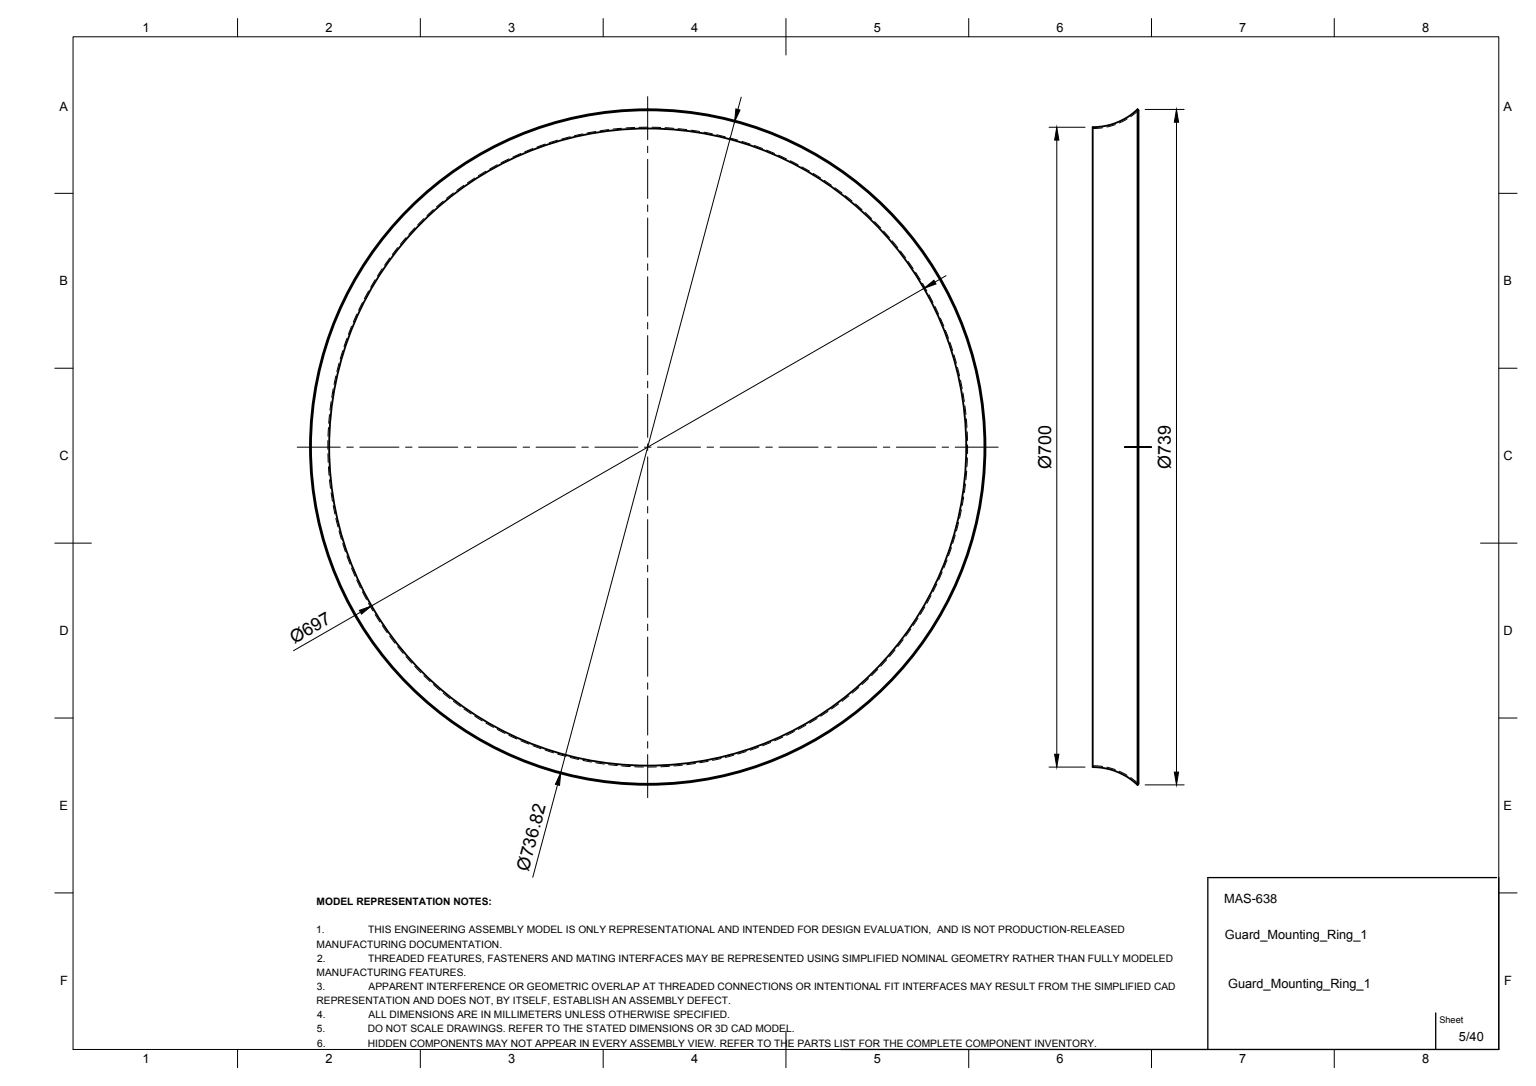
ISO-10303-21;
HEADER;
FILE_DESCRIPTION((''),'2;1');
FILE_NAME('Guard_Mounting_Ring_1.step','2026-10-09T12:00:21-07:00',(''),(''),'','','');
FILE_SCHEMA (('AUTOMOTIVE_DESIGN { 1 0 10303 214 3 1 1 }'));
ENDSEC;
DATA;
#10=MECHANICAL_DESIGN_GEOMETRIC_PRESENTATION_REPRESENTATION('',(#396),#10334);
#332=SHAPE_REPRESENTATION_RELATIONSHIP('SRR','None',#10448,#364) ;
#364=ADVANCED_BREP_SHAPE_REPRESENTATION('',(#436),#10300) ;
#396=STYLED_ITEM('',(#10631),#436) ;
#436=MANIFOLD_SOLID_BREP('Body1',#3558) ;
#468=FACE_BOUND('',#1054,.T.) ;
#477=PLANE('',#3957) ;
#532=LINE('',#5624,#690) ;
#690=VECTOR('',#4472,36.8410607518303) ;
#848=CONICAL_SURFACE('',#3956,36.8410607518303,0.812867971023228) ;
#851=FACE_OUTER_BOUND('',#1050,.T.) ;
#852=FACE_OUTER_BOUND('',#1051,.T.) ;
#853=FACE_OUTER_BOUND('',#1052,.T.) ;
#854=FACE_OUTER_BOUND('',#1053,.T.) ;
#1050=EDGE_LOOP('',(#2307,#2308,#2309,#2310,#2311)) ;
#1051=EDGE_LOOP('',(#2312,#2313,#2314,#2315,#2316)) ;
#1052=EDGE_LOOP('',(#2317,#2318,#2319,#2320,#2321,#2322)) ;
#1053=EDGE_LOOP('',(#2323)) ;
#1054=EDGE_LOOP('',(#2324)) ;
#1258=CIRCLE('',#3947,36.9499999999999) ;
#1259=CIRCLE('',#3948,36.9499999999999) ;
#1260=CIRCLE('',#3949,7.1235909466484) ;
#1261=CIRCLE('',#3950,35.) ;
#1262=CIRCLE('',#3952,34.8499999999999) ;
#1263=CIRCLE('',#3953,7.27359094664848) ;
#1264=CIRCLE('',#3954,36.8410607518303) ;
#1265=CIRCLE('',#3955,36.8410607518303) ;
#1499=VERTEX_POINT('',#5608) ;
#1500=VERTEX_POINT('',#5609) ;
#1501=VERTEX_POINT('',#5612) ;
#1502=VERTEX_POINT('',#5616) ;
#1503=VERTEX_POINT('',#5618) ;
#1504=VERTEX_POINT('',#5620) ;
#1810=EDGE_CURVE('',#1499,#1500,#1258,.T.) ;
#1811=EDGE_CURVE('',#1500,#1499,#1259,.T.) ;
#1812=EDGE_CURVE('',#1500,#1501,#1260,.T.) ;
#1813=EDGE_CURVE('',#1501,#1501,#1261,.T.) ;
#1814=EDGE_CURVE('',#1502,#1502,#1262,.T.) ;
#1815=EDGE_CURVE('',#1502,#1503,#1263,.T.) ;
#1816=EDGE_CURVE('',#1503,#1504,#1264,.T.) ;
#1817=EDGE_CURVE('',#1504,#1503,#1265,.T.) ;
#1818=EDGE_CURVE('',#1499,#1504,#532,.T.) ;
#2307=ORIENTED_EDGE('',*,*,#1810,.F.) ;
#2308=ORIENTED_EDGE('',*,*,#1811,.F.) ;
#2309=ORIENTED_EDGE('',*,*,#1812,.T.) ;
#2310=ORIENTED_EDGE('',*,*,#1813,.T.) ;
#2311=ORIENTED_EDGE('',*,*,#1812,.F.) ;
#2312=ORIENTED_EDGE('',*,*,#1814,.F.) ;
#2313=ORIENTED_EDGE('',*,*,#1815,.T.) ;
#2314=ORIENTED_EDGE('',*,*,#1816,.T.) ;
#2315=ORIENTED_EDGE('',*,*,#1817,.T.) ;
#2316=ORIENTED_EDGE('',*,*,#1815,.F.) ;
#2317=ORIENTED_EDGE('',*,*,#1810,.T.) ;
#2318=ORIENTED_EDGE('',*,*,#1811,.T.) ;
#2319=ORIENTED_EDGE('',*,*,#1818,.T.) ;
#2320=ORIENTED_EDGE('',*,*,#1816,.F.) ;
#2321=ORIENTED_EDGE('',*,*,#1817,.F.) ;
#2322=ORIENTED_EDGE('',*,*,#1818,.F.) ;
#2323=ORIENTED_EDGE('',*,*,#1813,.F.) ;
#2324=ORIENTED_EDGE('',*,*,#1814,.T.) ;
#3301=TOROIDAL_SURFACE('',#3946,42.1235909466484,7.1235909466484) ;
#3302=TOROIDAL_SURFACE('',#3951,42.1235909466484,7.27359094664848) ;
#3359=ADVANCED_FACE('',(#851),#3301,.F.) ;
#3360=ADVANCED_FACE('',(#852),#3302,.T.) ;
#3361=ADVANCED_FACE('',(#853),#848,.T.) ;
#3362=ADVANCED_FACE('',(#854,#468),#477,.F.) ;
#3558=CLOSED_SHELL('',(#3359,#3360,#3361,#3362)) ;
#3945=AXIS2_PLACEMENT_3D('',#5606,#4448,#4449) ;
#3946=AXIS2_PLACEMENT_3D('',#5607,#4450,#4451) ;
#3947=AXIS2_PLACEMENT_3D('',#5610,#4452,#4453) ;
#3948=AXIS2_PLACEMENT_3D('',#5611,#4454,#4455) ;
#3949=AXIS2_PLACEMENT_3D('',#5613,#4456,#4457) ;
#3950=AXIS2_PLACEMENT_3D('',#5614,#4458,#4459) ;
#3951=AXIS2_PLACEMENT_3D('',#5615,#4460,#4461) ;
#3952=AXIS2_PLACEMENT_3D('',#5617,#4462,#4463) ;
#3953=AXIS2_PLACEMENT_3D('',#5619,#4464,#4465) ;
#3954=AXIS2_PLACEMENT_3D('',#5621,#4466,#4467) ;
#3955=AXIS2_PLACEMENT_3D('',#5622,#4468,#4469) ;
#3956=AXIS2_PLACEMENT_3D('',#5623,#4470,#4471) ;
#3957=AXIS2_PLACEMENT_3D('',#5625,#4473,#4474) ;
#4448=DIRECTION('axis',(0.,0.,1.)) ;
#4449=DIRECTION('refdir',(1.,0.,0.)) ;
#4450=DIRECTION('center_axis',(0.,-1.,0.)) ;
#4451=DIRECTION('ref_axis',(0.,0.,-1.)) ;
#4452=DIRECTION('center_axis',(0.,-1.,0.)) ;
#4453=DIRECTION('ref_axis',(0.,0.,-1.)) ;
#4454=DIRECTION('center_axis',(0.,-1.,0.)) ;
#4455=DIRECTION('ref_axis',(0.,0.,-1.)) ;
#4456=DIRECTION('center_axis',(1.,0.,1.44280892518809E-16)) ;
#4457=DIRECTION('ref_axis',(-1.44280892518809E-16,0.,1.)) ;
#4458=DIRECTION('center_axis',(0.,-1.,0.)) ;
#4459=DIRECTION('ref_axis',(0.,0.,-1.)) ;
#4460=DIRECTION('center_axis',(0.,-1.,0.)) ;
#4461=DIRECTION('ref_axis',(0.,0.,-1.)) ;
#4462=DIRECTION('center_axis',(0.,-1.,0.)) ;
#4463=DIRECTION('ref_axis',(0.,0.,-1.)) ;
#4464=DIRECTION('center_axis',(-1.,0.,-1.43842767649164E-16)) ;
#4465=DIRECTION('ref_axis',(-1.43842767649164E-16,0.,1.)) ;
#4466=DIRECTION('center_axis',(0.,-1.,0.)) ;
#4467=DIRECTION('ref_axis',(0.,0.,-1.)) ;
#4468=DIRECTION('center_axis',(0.,-1.,0.)) ;
#4469=DIRECTION('ref_axis',(0.,0.,-1.)) ;
#4470=DIRECTION('center_axis',(0.,1.,0.)) ;
#4471=DIRECTION('ref_axis',(0.,0.,1.)) ;
#4472=DIRECTION('',(8.89414010481862E-17,-0.687418365521554,0.726261654463235)) ;
#4473=DIRECTION('center_axis',(0.,-1.,0.)) ;
#4474=DIRECTION('ref_axis',(0.,0.,-1.)) ;
#5606=CARTESIAN_POINT('',(0.,0.,0.)) ;
#5607=CARTESIAN_POINT('Origin',(23.47768801576,48.8830586252741,68.2224337400009)) ;
#5608=CARTESIAN_POINT('',(23.47768801576,43.9861713801022,31.272433740001)) ;
#5609=CARTESIAN_POINT('',(23.47768801576,43.9861713801022,105.172433740001)) ;
#5610=CARTESIAN_POINT('Origin',(23.47768801576,43.9861713801022,68.2224337400009)) ;
#5611=CARTESIAN_POINT('Origin',(23.47768801576,43.9861713801022,68.2224337400009)) ;
#5612=CARTESIAN_POINT('',(23.4776880157599,48.8830586252741,103.222433740001)) ;
#5613=CARTESIAN_POINT('Origin',(23.47768801576,48.8830586252741,110.346024686649)) ;
#5614=CARTESIAN_POINT('Origin',(23.47768801576,48.8830586252741,68.2224337400009)) ;
#5615=CARTESIAN_POINT('Origin',(23.47768801576,48.8830586252741,68.2224337400009)) ;
#5616=CARTESIAN_POINT('',(23.4776880157599,48.8830586252741,103.072433740001)) ;
#5617=CARTESIAN_POINT('Origin',(23.47768801576,48.8830586252741,68.2224337400009)) ;
#5618=CARTESIAN_POINT('',(23.47768801576,43.8830586252739,105.063494491831)) ;
#5619=CARTESIAN_POINT('Origin',(23.47768801576,48.8830586252741,110.346024686649)) ;
#5620=CARTESIAN_POINT('',(23.47768801576,43.8830586252739,31.3813729881705)) ;
#5621=CARTESIAN_POINT('Origin',(23.47768801576,43.8830586252739,68.2224337400009)) ;
#5622=CARTESIAN_POINT('Origin',(23.47768801576,43.8830586252739,68.2224337400009)) ;
#5623=CARTESIAN_POINT('Origin',(23.47768801576,43.8830586252739,68.2224337400009)) ;
#5624=CARTESIAN_POINT('',(23.47768801576,43.8830586252739,31.3813729881706)) ;
#5625=CARTESIAN_POINT('Origin',(58.3276880157596,48.8830586252741,68.2224337400009)) ;
#10263=UNCERTAINTY_MEASURE_WITH_UNIT(LENGTH_MEASURE(0.001),#10335,
'DISTANCE_ACCURACY_VALUE',
'Maximum model space distance between geometric entities at asserted c
onnectivities') ;
#10297=UNCERTAINTY_MEASURE_WITH_UNIT(LENGTH_MEASURE(0.001),#10335,
'DISTANCE_ACCURACY_VALUE',
'Maximum model space distance between geometric entities at asserted c
onnectivities') ;
#10300=(
GEOMETRIC_REPRESENTATION_CONTEXT(3)
GLOBAL_UNCERTAINTY_ASSIGNED_CONTEXT((#10263))
GLOBAL_UNIT_ASSIGNED_CONTEXT((#10335,#10337,#10338))
REPRESENTATION_CONTEXT('','3D')
) ;
#10334=(
GEOMETRIC_REPRESENTATION_CONTEXT(3)
GLOBAL_UNCERTAINTY_ASSIGNED_CONTEXT((#10297))
GLOBAL_UNIT_ASSIGNED_CONTEXT((#10335,#10337,#10338))
REPRESENTATION_CONTEXT('','3D')
) ;
#10335=(
LENGTH_UNIT()
NAMED_UNIT(*)
SI_UNIT(.CENTI.,.METRE.)
) ;
#10337=(
NAMED_UNIT(*)
PLANE_ANGLE_UNIT()
SI_UNIT($,.RADIAN.)
) ;
#10338=(
NAMED_UNIT(*)
SI_UNIT($,.STERADIAN.)
SOLID_ANGLE_UNIT()
) ;
#10341=SHAPE_DEFINITION_REPRESENTATION(#10377,#10448) ;
#10377=PRODUCT_DEFINITION_SHAPE('',$,#10485) ;
#10448=SHAPE_REPRESENTATION('',(#3945),#10300) ;
#10482=PRODUCT_DEFINITION_CONTEXT('part definition',#10592,'design') ;
#10485=PRODUCT_DEFINITION('Guard_Mounting_Ring_1',
'Guard_Mounting_Ring_1',#10521,#10482) ;
#10521=PRODUCT_DEFINITION_FORMATION('',$,#10596) ;
#10592=APPLICATION_CONTEXT(
'Core Data for Automotive Mechanical Design Process') ;
#10593=PRODUCT_CONTEXT('part definition',#10592,'mechanical') ;
#10596=PRODUCT('Guard_Mounting_Ring_1','Guard_Mounting_Ring_1',$,(#10593)) ;
#10631=PRESENTATION_STYLE_ASSIGNMENT((#10635)) ;
#10635=SURFACE_STYLE_USAGE(.BOTH.,#10639) ;
#10639=SURFACE_SIDE_STYLE('',(#10643)) ;
#10643=SURFACE_STYLE_FILL_AREA(#10647) ;
#10647=FILL_AREA_STYLE('Opaque(25,25,25)',(#10651)) ;
#10651=FILL_AREA_STYLE_COLOUR('Opaque(25,25,25)',#10655) ;
#10655=COLOUR_RGB('Opaque(25,25,25)', 0.09019608, 0.27058824, 0.51372549) ;
ENDSEC;
END-ISO-10303-21;
